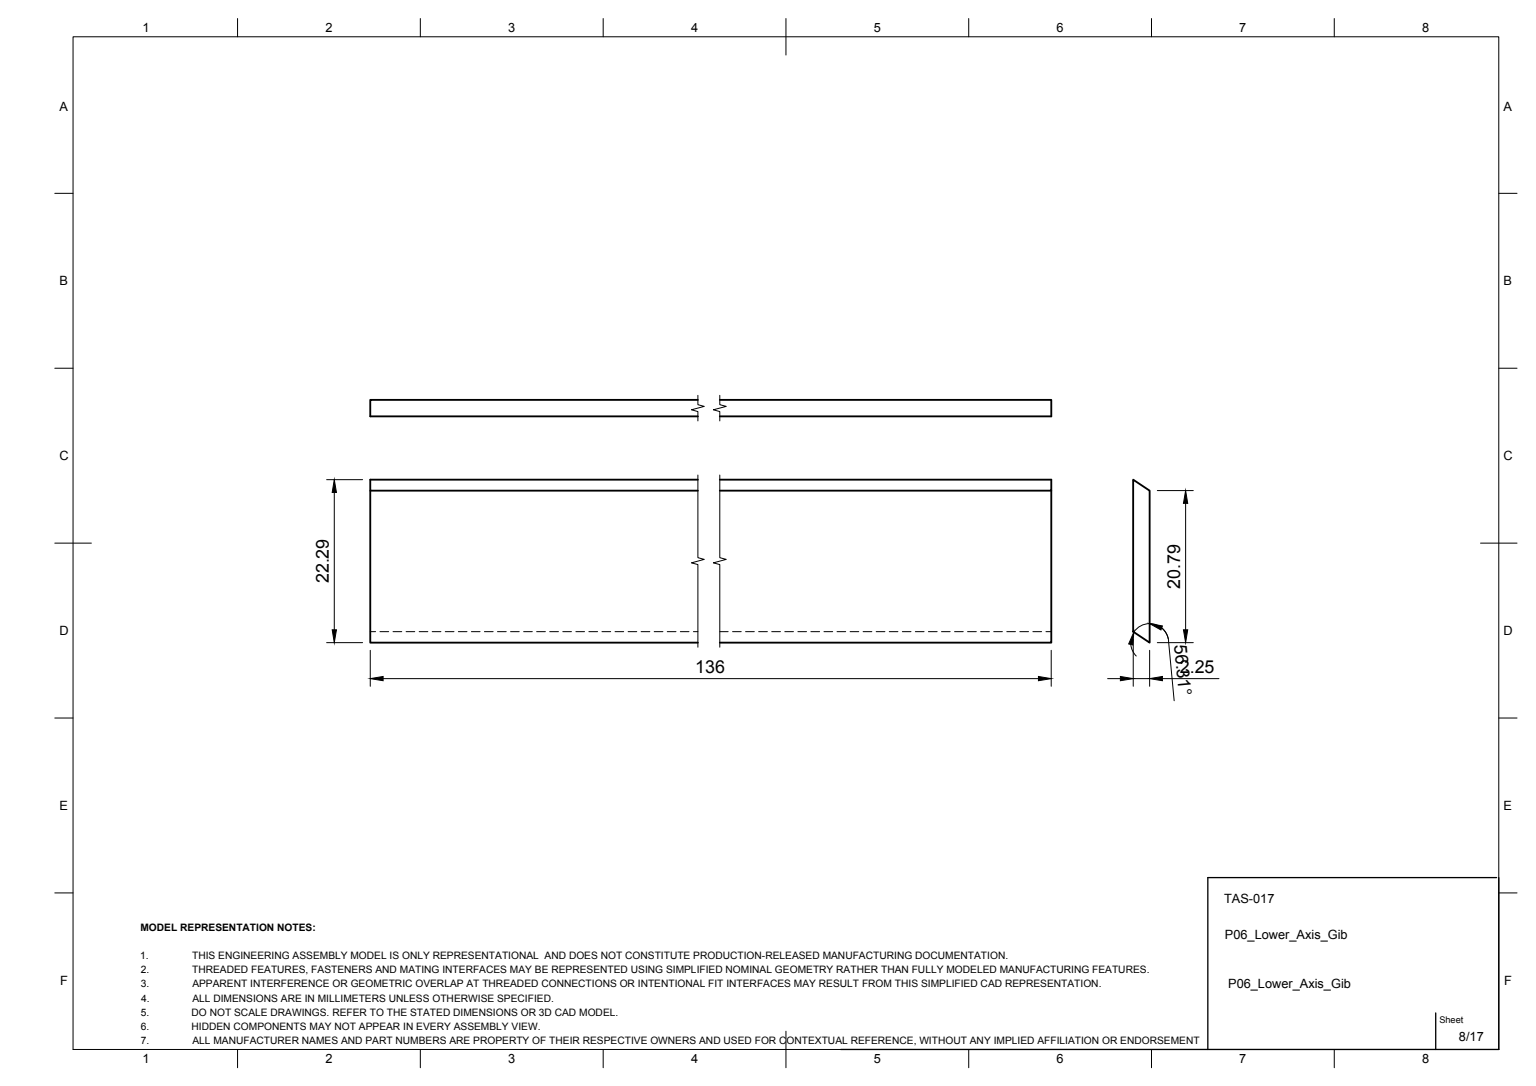
ISO-10303-21;
HEADER;
/* Generated by software containing ST-Developer
 * from STEP Tools, Inc. (www.steptools.com) 
 */

FILE_DESCRIPTION(
/* description */ ('STEP AP203'),
/* implementation_level */ '2;1');

FILE_NAME(
/* name */ 'P06_Lower_Axis_Gib.step',
/* time_stamp */ '2026-11-15T15:04:01-08:00',
/* author */ (''),
/* organization */ (''),
/* preprocessor_version */ 'ST-DEVELOPER v20.2',
/* originating_system */ 'Autodesk Translation Framework v15.17.0.0',
/* authorisation */ '');

FILE_SCHEMA (('AUTOMOTIVE_DESIGN { 1 0 10303 214 3 1 1 }'));
ENDSEC;

DATA;
#10=MECHANICAL_DESIGN_GEOMETRIC_PRESENTATION_REPRESENTATION('',(#286),#16598);
#208=SHAPE_REPRESENTATION_RELATIONSHIP('SRR','None',#16702,#232);
#232=ADVANCED_BREP_SHAPE_REPRESENTATION('',(#256),#16578);
#256=MANIFOLD_SOLID_BREP('Body1',#9791);
#286=STYLED_ITEM('',(#16827),#256);
#575=PLANE('',#10300);
#576=PLANE('',#10301);
#577=PLANE('',#10302);
#578=PLANE('',#10303);
#579=PLANE('',#10304);
#580=PLANE('',#10305);
#1077=FACE_OUTER_BOUND('',#1658,.T.);
#1078=FACE_OUTER_BOUND('',#1659,.T.);
#1079=FACE_OUTER_BOUND('',#1660,.T.);
#1080=FACE_OUTER_BOUND('',#1661,.T.);
#1081=FACE_OUTER_BOUND('',#1662,.T.);
#1082=FACE_OUTER_BOUND('',#1663,.T.);
#1658=EDGE_LOOP('',(#7461,#7462,#7463,#7464));
#1659=EDGE_LOOP('',(#7465,#7466,#7467,#7468));
#1660=EDGE_LOOP('',(#7469,#7470,#7471,#7472));
#1661=EDGE_LOOP('',(#7473,#7474,#7475,#7476));
#1662=EDGE_LOOP('',(#7477,#7478,#7479,#7480));
#1663=EDGE_LOOP('',(#7481,#7482,#7483,#7484));
#2516=LINE('',#14575,#3564);
#2517=LINE('',#14577,#3565);
#2518=LINE('',#14579,#3566);
#2519=LINE('',#14580,#3567);
#2520=LINE('',#14583,#3568);
#2521=LINE('',#14585,#3569);
#2522=LINE('',#14586,#3570);
#2523=LINE('',#14589,#3571);
#2524=LINE('',#14591,#3572);
#2525=LINE('',#14592,#3573);
#2526=LINE('',#14594,#3574);
#2527=LINE('',#14595,#3575);
#3564=VECTOR('',#11758,1000.);
#3565=VECTOR('',#11759,1000.);
#3566=VECTOR('',#11760,1000.);
#3567=VECTOR('',#11761,1000.);
#3568=VECTOR('',#11764,1000.);
#3569=VECTOR('',#11765,1000.);
#3570=VECTOR('',#11766,1000.);
#3571=VECTOR('',#11769,1000.);
#3572=VECTOR('',#11770,1000.);
#3573=VECTOR('',#11771,1000.);
#3574=VECTOR('',#11774,1000.);
#3575=VECTOR('',#11775,1000.);
#4743=VERTEX_POINT('',#14573);
#4744=VERTEX_POINT('',#14574);
#4745=VERTEX_POINT('',#14576);
#4746=VERTEX_POINT('',#14578);
#4747=VERTEX_POINT('',#14582);
#4748=VERTEX_POINT('',#14584);
#4749=VERTEX_POINT('',#14588);
#4750=VERTEX_POINT('',#14590);
#5743=EDGE_CURVE('',#4743,#4744,#2516,.T.);
#5744=EDGE_CURVE('',#4745,#4744,#2517,.T.);
#5745=EDGE_CURVE('',#4746,#4745,#2518,.T.);
#5746=EDGE_CURVE('',#4746,#4743,#2519,.T.);
#5747=EDGE_CURVE('',#4744,#4747,#2520,.T.);
#5748=EDGE_CURVE('',#4748,#4747,#2521,.T.);
#5749=EDGE_CURVE('',#4745,#4748,#2522,.T.);
#5750=EDGE_CURVE('',#4747,#4749,#2523,.T.);
#5751=EDGE_CURVE('',#4750,#4749,#2524,.T.);
#5752=EDGE_CURVE('',#4748,#4750,#2525,.T.);
#5753=EDGE_CURVE('',#4749,#4743,#2526,.T.);
#5754=EDGE_CURVE('',#4750,#4746,#2527,.T.);
#7461=ORIENTED_EDGE('',*,*,#5743,.T.);
#7462=ORIENTED_EDGE('',*,*,#5744,.F.);
#7463=ORIENTED_EDGE('',*,*,#5745,.F.);
#7464=ORIENTED_EDGE('',*,*,#5746,.T.);
#7465=ORIENTED_EDGE('',*,*,#5747,.T.);
#7466=ORIENTED_EDGE('',*,*,#5748,.F.);
#7467=ORIENTED_EDGE('',*,*,#5749,.F.);
#7468=ORIENTED_EDGE('',*,*,#5744,.T.);
#7469=ORIENTED_EDGE('',*,*,#5750,.T.);
#7470=ORIENTED_EDGE('',*,*,#5751,.F.);
#7471=ORIENTED_EDGE('',*,*,#5752,.F.);
#7472=ORIENTED_EDGE('',*,*,#5748,.T.);
#7473=ORIENTED_EDGE('',*,*,#5753,.T.);
#7474=ORIENTED_EDGE('',*,*,#5746,.F.);
#7475=ORIENTED_EDGE('',*,*,#5754,.F.);
#7476=ORIENTED_EDGE('',*,*,#5751,.T.);
#7477=ORIENTED_EDGE('',*,*,#5745,.T.);
#7478=ORIENTED_EDGE('',*,*,#5749,.T.);
#7479=ORIENTED_EDGE('',*,*,#5752,.T.);
#7480=ORIENTED_EDGE('',*,*,#5754,.T.);
#7481=ORIENTED_EDGE('',*,*,#5743,.F.);
#7482=ORIENTED_EDGE('',*,*,#5753,.F.);
#7483=ORIENTED_EDGE('',*,*,#5750,.F.);
#7484=ORIENTED_EDGE('',*,*,#5747,.F.);
#9402=ADVANCED_FACE('',(#1077),#575,.F.);
#9403=ADVANCED_FACE('',(#1078),#576,.F.);
#9404=ADVANCED_FACE('',(#1079),#577,.F.);
#9405=ADVANCED_FACE('',(#1080),#578,.F.);
#9406=ADVANCED_FACE('',(#1081),#579,.T.);
#9407=ADVANCED_FACE('',(#1082),#580,.F.);
#9791=CLOSED_SHELL('',(#9402,#9403,#9404,#9405,#9406,#9407));
#10299=AXIS2_PLACEMENT_3D('',#14571,#11754,#11755);
#10300=AXIS2_PLACEMENT_3D('',#14572,#11756,#11757);
#10301=AXIS2_PLACEMENT_3D('',#14581,#11762,#11763);
#10302=AXIS2_PLACEMENT_3D('',#14587,#11767,#11768);
#10303=AXIS2_PLACEMENT_3D('',#14593,#11772,#11773);
#10304=AXIS2_PLACEMENT_3D('',#14596,#11776,#11777);
#10305=AXIS2_PLACEMENT_3D('',#14597,#11778,#11779);
#11754=DIRECTION('axis',(0.,0.,1.));
#11755=DIRECTION('refdir',(1.,0.,0.));
#11756=DIRECTION('center_axis',(0.,0.83205103426688,-0.55469908633007));
#11757=DIRECTION('ref_axis',(0.,0.55469908633007,0.83205103426688));
#11758=DIRECTION('',(0.,-0.55469908633007,-0.83205103426688));
#11759=DIRECTION('',(-1.,0.,0.));
#11760=DIRECTION('',(0.,-0.55469908633007,-0.83205103426688));
#11761=DIRECTION('',(-1.,0.,0.));
#11762=DIRECTION('center_axis',(0.,0.,1.));
#11763=DIRECTION('ref_axis',(1.,0.,0.));
#11764=DIRECTION('',(0.,1.,0.));
#11765=DIRECTION('',(-1.,0.,0.));
#11766=DIRECTION('',(0.,1.,0.));
#11767=DIRECTION('center_axis',(0.,-0.83205103426688,0.55469908633007));
#11768=DIRECTION('ref_axis',(0.,-0.55469908633007,-0.83205103426688));
#11769=DIRECTION('',(0.,0.55469908633007,0.83205103426688));
#11770=DIRECTION('',(-1.,0.,0.));
#11771=DIRECTION('',(0.,0.55469908633007,0.83205103426688));
#11772=DIRECTION('center_axis',(0.,0.,-1.));
#11773=DIRECTION('ref_axis',(-1.,0.,0.));
#11774=DIRECTION('',(0.,-1.,0.));
#11775=DIRECTION('',(0.,-1.,0.));
#11776=DIRECTION('center_axis',(1.,0.,0.));
#11777=DIRECTION('ref_axis',(0.,0.,-1.));
#11778=DIRECTION('center_axis',(1.,0.,0.));
#11779=DIRECTION('ref_axis',(0.,0.,-1.));
#14571=CARTESIAN_POINT('',(0.,0.,0.));
#14572=CARTESIAN_POINT('Origin',(68.,45.2333,33.9));
#14573=CARTESIAN_POINT('',(-68.,45.2333,33.9));
#14574=CARTESIAN_POINT('',(-68.,33.7,16.6));
#14575=CARTESIAN_POINT('',(-68.,45.2333,33.9));
#14576=CARTESIAN_POINT('',(68.,33.7,16.6));
#14577=CARTESIAN_POINT('',(68.,33.7,16.6));
#14578=CARTESIAN_POINT('',(68.,45.2333,33.9));
#14579=CARTESIAN_POINT('',(68.,45.2333,33.9));
#14580=CARTESIAN_POINT('',(68.,45.2333,33.9));
#14581=CARTESIAN_POINT('Origin',(68.,33.7,16.6));
#14582=CARTESIAN_POINT('',(-68.,36.4,16.6));
#14583=CARTESIAN_POINT('',(-68.,33.7,16.6));
#14584=CARTESIAN_POINT('',(68.,36.4,16.6));
#14585=CARTESIAN_POINT('',(68.,36.4,16.6));
#14586=CARTESIAN_POINT('',(68.,33.7,16.6));
#14587=CARTESIAN_POINT('Origin',(68.,36.4,16.6));
#14588=CARTESIAN_POINT('',(-68.,47.9333,33.9));
#14589=CARTESIAN_POINT('',(-68.,36.4,16.6));
#14590=CARTESIAN_POINT('',(68.,47.9333,33.9));
#14591=CARTESIAN_POINT('',(68.,47.9333,33.9));
#14592=CARTESIAN_POINT('',(68.,36.4,16.6));
#14593=CARTESIAN_POINT('Origin',(68.,47.9333,33.9));
#14594=CARTESIAN_POINT('',(-68.,47.9333,33.9));
#14595=CARTESIAN_POINT('',(68.,47.9333,33.9));
#14596=CARTESIAN_POINT('Origin',(68.,0.,0.));
#14597=CARTESIAN_POINT('Origin',(-68.,0.,0.));
#16552=UNCERTAINTY_MEASURE_WITH_UNIT(LENGTH_MEASURE(0.01),#16599,
'DISTANCE_ACCURACY_VALUE',
'Maximum model space distance between geometric entities at asserted c
onnectivities');
#16572=UNCERTAINTY_MEASURE_WITH_UNIT(LENGTH_MEASURE(0.01),#16599,
'DISTANCE_ACCURACY_VALUE',
'Maximum model space distance between geometric entities at asserted c
onnectivities');
#16578=(
GEOMETRIC_REPRESENTATION_CONTEXT(3)
GLOBAL_UNCERTAINTY_ASSIGNED_CONTEXT((#16552))
GLOBAL_UNIT_ASSIGNED_CONTEXT((#16599,#16601,#16602))
REPRESENTATION_CONTEXT('','3D')
);
#16598=(
GEOMETRIC_REPRESENTATION_CONTEXT(3)
GLOBAL_UNCERTAINTY_ASSIGNED_CONTEXT((#16572))
GLOBAL_UNIT_ASSIGNED_CONTEXT((#16599,#16601,#16602))
REPRESENTATION_CONTEXT('','3D')
);
#16599=(
LENGTH_UNIT()
NAMED_UNIT(*)
SI_UNIT(.MILLI.,.METRE.)
);
#16601=(
NAMED_UNIT(*)
PLANE_ANGLE_UNIT()
SI_UNIT($,.RADIAN.)
);
#16602=(
NAMED_UNIT(*)
SI_UNIT($,.STERADIAN.)
SOLID_ANGLE_UNIT()
);
#16608=SHAPE_DEFINITION_REPRESENTATION(#16633,#16702);
#16633=PRODUCT_DEFINITION_SHAPE('',$,#16728);
#16702=SHAPE_REPRESENTATION('',(#10299),#16578);
#16722=PRODUCT_DEFINITION_CONTEXT('part definition',#16799,'design');
#16728=PRODUCT_DEFINITION('P06_Lower_Axis_Gib','P06_Lower_Axis_Gib',#16753,
#16722);
#16753=PRODUCT_DEFINITION_FORMATION('',$,#16806);
#16799=APPLICATION_CONTEXT(
'Core Data for Automotive Mechanical Design Process');
#16800=PRODUCT_CONTEXT('part definition',#16799,'mechanical');
#16806=PRODUCT('P06_Lower_Axis_Gib','P06_Lower_Axis_Gib',$,(#16800));
#16827=PRESENTATION_STYLE_ASSIGNMENT((#16836));
#16836=SURFACE_STYLE_USAGE(.BOTH.,#16845);
#16845=SURFACE_SIDE_STYLE('',(#16854));
#16854=SURFACE_STYLE_FILL_AREA(#16863);
#16863=FILL_AREA_STYLE('Gray',(#16872));
#16872=FILL_AREA_STYLE_COLOUR('Gray',#16881);
#16881=COLOUR_RGB('Gray',0.501960784313725,0.501960784313725,0.501960784313725);
ENDSEC;
END-ISO-10303-21;
